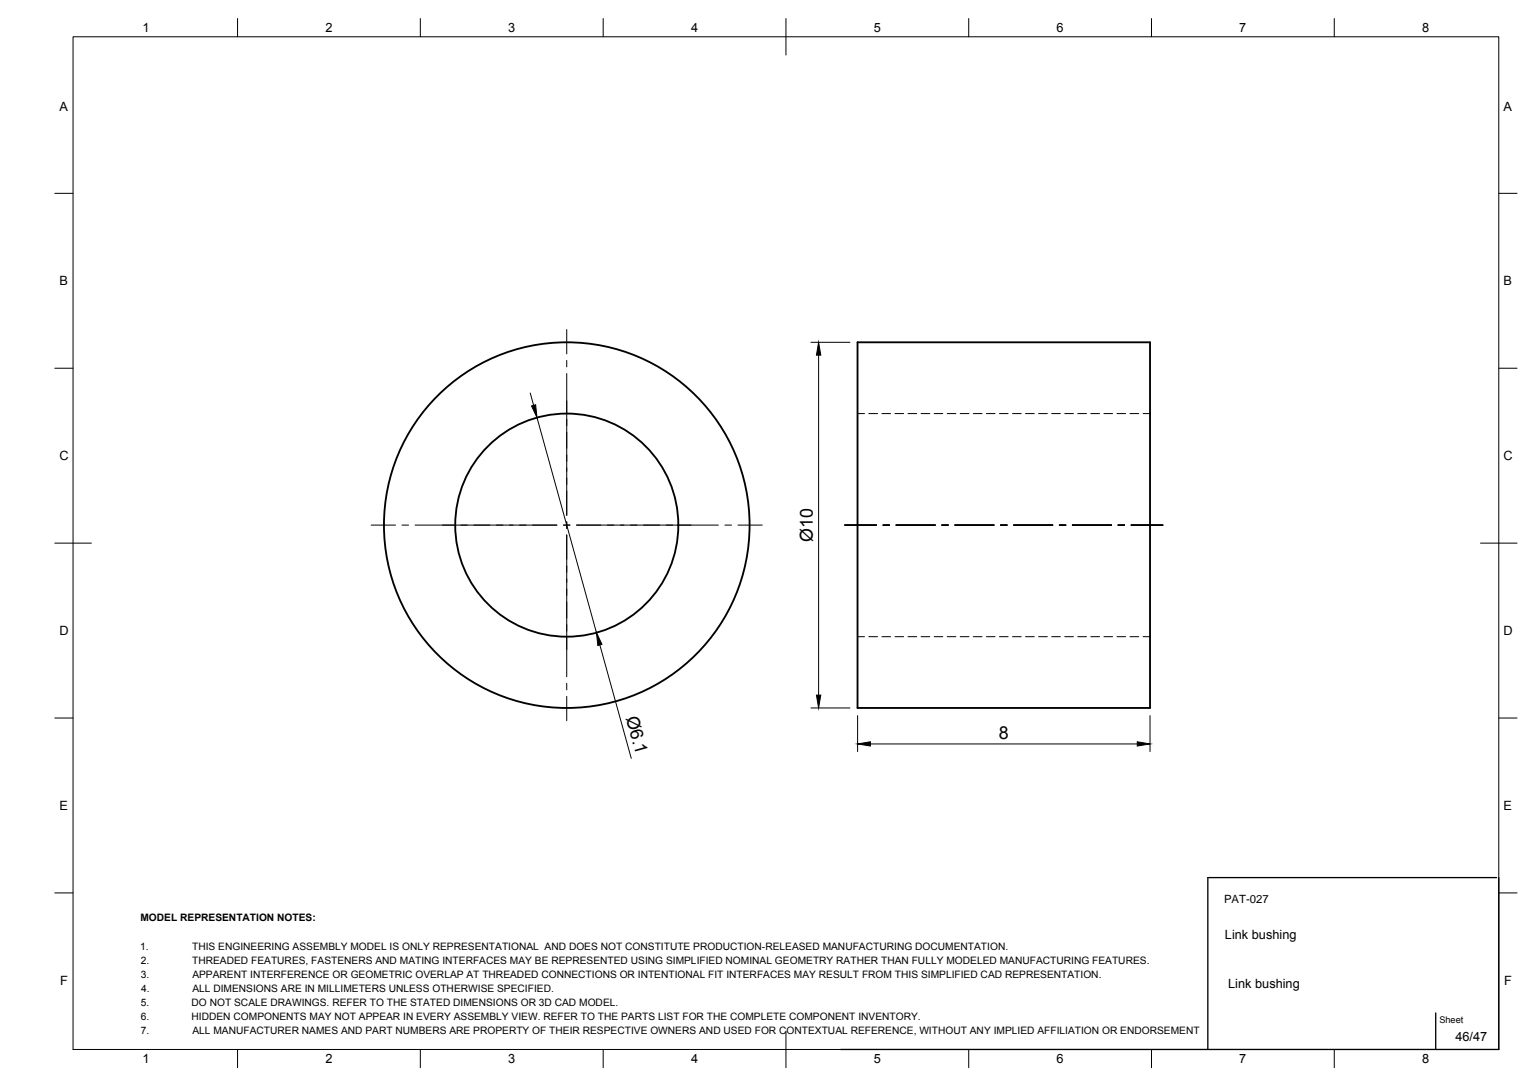
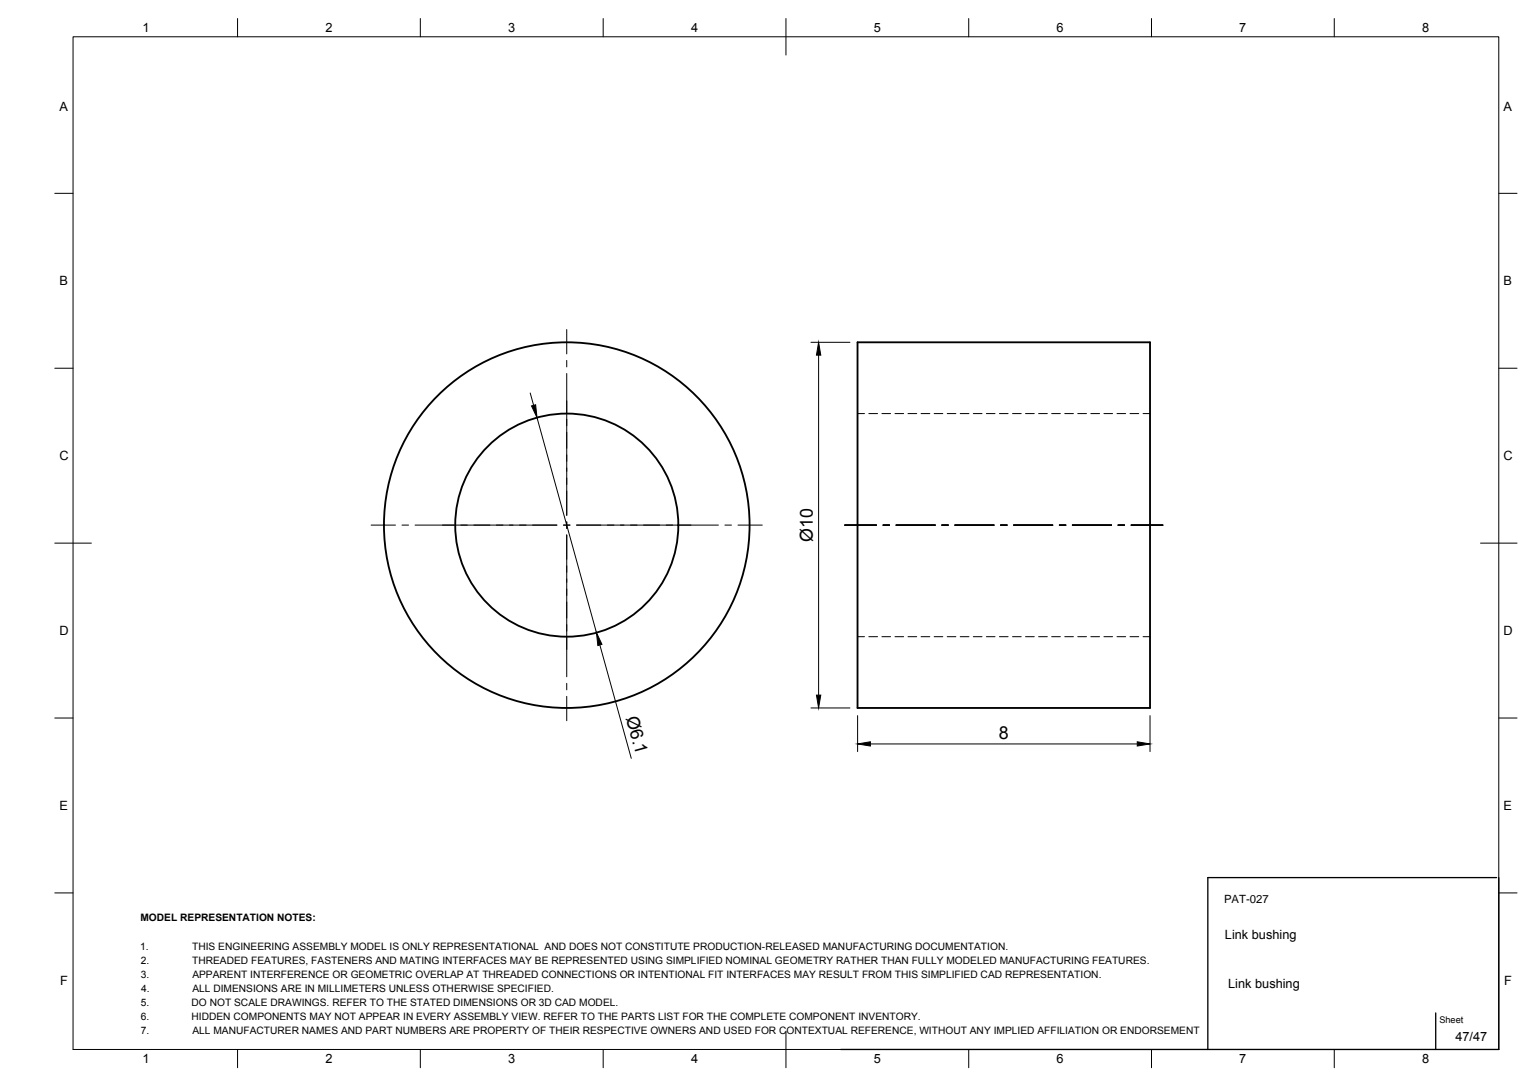
ISO-10303-21;
HEADER;
/* Generated by software containing ST-Developer
 * from STEP Tools, Inc. (www.steptools.com) 
 */

FILE_DESCRIPTION(
/* description */ ('Crank-driven oscillating fan base (mechanism only)'),

/* implementation_level */ '2;1');

FILE_NAME(
/* name */ 'Link bushing.step',
/* time_stamp */ '2026-10-28T03:25:00-07:00',
/* author */ (''),
/* organization */ (''),
/* preprocessor_version */ 'ST-DEVELOPER v20.2',
/* originating_system */ 'Autodesk Translation Framework v15.17.0.0',
/* authorisation */ '');

FILE_SCHEMA (('AUTOMOTIVE_DESIGN { 1 0 10303 214 3 1 1 }'));
ENDSEC;

DATA;
#10=MECHANICAL_DESIGN_GEOMETRIC_PRESENTATION_REPRESENTATION('',(#483),#11916);
#395=SHAPE_REPRESENTATION_RELATIONSHIP('SRR','None',#12123,#435);
#435=ADVANCED_BREP_SHAPE_REPRESENTATION('',(#528),#11914);
#483=STYLED_ITEM('',(#12361),#528);
#528=MANIFOLD_SOLID_BREP('Body1',#6116);
#688=FACE_BOUND('',#1789,.T.);
#689=FACE_BOUND('',#1791,.T.);
#882=PLANE('',#7393);
#883=PLANE('',#7394);
#1253=FACE_OUTER_BOUND('',#1786,.T.);
#1254=FACE_OUTER_BOUND('',#1787,.T.);
#1255=FACE_OUTER_BOUND('',#1788,.T.);
#1256=FACE_OUTER_BOUND('',#1790,.T.);
#1786=EDGE_LOOP('',(#5522,#5523,#5524,#5525));
#1787=EDGE_LOOP('',(#5526,#5527,#5528,#5529));
#1788=EDGE_LOOP('',(#5530));
#1789=EDGE_LOOP('',(#5531));
#1790=EDGE_LOOP('',(#5532));
#1791=EDGE_LOOP('',(#5533));
#2127=LINE('',#11791,#2460);
#2128=LINE('',#11797,#2461);
#2460=VECTOR('',#9400,0.305);
#2461=VECTOR('',#9407,0.5);
#2821=CIRCLE('',#7388,0.305);
#2822=CIRCLE('',#7389,0.305);
#2823=CIRCLE('',#7391,0.5);
#2824=CIRCLE('',#7392,0.5);
#3321=VERTEX_POINT('',#11788);
#3322=VERTEX_POINT('',#11790);
#3323=VERTEX_POINT('',#11794);
#3324=VERTEX_POINT('',#11796);
#4056=EDGE_CURVE('',#3321,#3321,#2821,.T.);
#4057=EDGE_CURVE('',#3321,#3322,#2127,.T.);
#4058=EDGE_CURVE('',#3322,#3322,#2822,.T.);
#4059=EDGE_CURVE('',#3323,#3323,#2823,.T.);
#4060=EDGE_CURVE('',#3323,#3324,#2128,.T.);
#4061=EDGE_CURVE('',#3324,#3324,#2824,.T.);
#5522=ORIENTED_EDGE('',*,*,#4056,.F.);
#5523=ORIENTED_EDGE('',*,*,#4057,.T.);
#5524=ORIENTED_EDGE('',*,*,#4058,.T.);
#5525=ORIENTED_EDGE('',*,*,#4057,.F.);
#5526=ORIENTED_EDGE('',*,*,#4059,.F.);
#5527=ORIENTED_EDGE('',*,*,#4060,.T.);
#5528=ORIENTED_EDGE('',*,*,#4061,.T.);
#5529=ORIENTED_EDGE('',*,*,#4060,.F.);
#5530=ORIENTED_EDGE('',*,*,#4059,.T.);
#5531=ORIENTED_EDGE('',*,*,#4056,.T.);
#5532=ORIENTED_EDGE('',*,*,#4061,.F.);
#5533=ORIENTED_EDGE('',*,*,#4058,.F.);
#5688=CYLINDRICAL_SURFACE('',#7387,0.305);
#5689=CYLINDRICAL_SURFACE('',#7390,0.5);
#6059=ADVANCED_FACE('',(#1253),#5688,.F.);
#6060=ADVANCED_FACE('',(#1254),#5689,.T.);
#6061=ADVANCED_FACE('',(#1255,#688),#882,.T.);
#6062=ADVANCED_FACE('',(#1256,#689),#883,.F.);
#6116=CLOSED_SHELL('',(#6059,#6060,#6061,#6062));
#7386=AXIS2_PLACEMENT_3D('',#11786,#9394,#9395);
#7387=AXIS2_PLACEMENT_3D('',#11787,#9396,#9397);
#7388=AXIS2_PLACEMENT_3D('',#11789,#9398,#9399);
#7389=AXIS2_PLACEMENT_3D('',#11792,#9401,#9402);
#7390=AXIS2_PLACEMENT_3D('',#11793,#9403,#9404);
#7391=AXIS2_PLACEMENT_3D('',#11795,#9405,#9406);
#7392=AXIS2_PLACEMENT_3D('',#11798,#9408,#9409);
#7393=AXIS2_PLACEMENT_3D('',#11799,#9410,#9411);
#7394=AXIS2_PLACEMENT_3D('',#11800,#9412,#9413);
#9394=DIRECTION('axis',(0.,0.,1.));
#9395=DIRECTION('refdir',(1.,0.,0.));
#9396=DIRECTION('center_axis',(0.,0.,1.));
#9397=DIRECTION('ref_axis',(1.,0.,0.));
#9398=DIRECTION('center_axis',(0.,0.,-1.));
#9399=DIRECTION('ref_axis',(1.,0.,0.));
#9400=DIRECTION('',(0.,0.,-1.));
#9401=DIRECTION('center_axis',(0.,0.,-1.));
#9402=DIRECTION('ref_axis',(1.,0.,0.));
#9403=DIRECTION('center_axis',(0.,0.,1.));
#9404=DIRECTION('ref_axis',(1.,0.,0.));
#9405=DIRECTION('center_axis',(0.,0.,1.));
#9406=DIRECTION('ref_axis',(1.,0.,0.));
#9407=DIRECTION('',(0.,0.,-1.));
#9408=DIRECTION('center_axis',(0.,0.,1.));
#9409=DIRECTION('ref_axis',(1.,0.,0.));
#9410=DIRECTION('center_axis',(0.,0.,1.));
#9411=DIRECTION('ref_axis',(1.,0.,0.));
#9412=DIRECTION('center_axis',(0.,0.,1.));
#9413=DIRECTION('ref_axis',(1.,0.,0.));
#11786=CARTESIAN_POINT('',(0.,0.,0.));
#11787=CARTESIAN_POINT('Origin',(-0.429855350392604,2.61349944954989,8.6));
#11788=CARTESIAN_POINT('',(-0.734855350392604,2.61349944954989,9.4));
#11789=CARTESIAN_POINT('Origin',(-0.429855350392604,2.61349944954989,9.4));
#11790=CARTESIAN_POINT('',(-0.734855350392604,2.61349944954989,8.6));
#11791=CARTESIAN_POINT('',(-0.734855350392604,2.61349944954989,8.6));
#11792=CARTESIAN_POINT('Origin',(-0.429855350392604,2.61349944954989,8.6));
#11793=CARTESIAN_POINT('Origin',(-0.429855350392604,2.61349944954989,8.6));
#11794=CARTESIAN_POINT('',(-0.929855350392604,2.61349944954989,9.4));
#11795=CARTESIAN_POINT('Origin',(-0.429855350392604,2.61349944954989,9.4));
#11796=CARTESIAN_POINT('',(-0.929855350392604,2.61349944954989,8.6));
#11797=CARTESIAN_POINT('',(-0.929855350392604,2.61349944954989,8.6));
#11798=CARTESIAN_POINT('Origin',(-0.429855350392604,2.61349944954989,8.6));
#11799=CARTESIAN_POINT('Origin',(-0.429855350392604,2.61349944954989,9.4));
#11800=CARTESIAN_POINT('Origin',(-0.429855350392604,2.61349944954989,8.6));
#11867=UNCERTAINTY_MEASURE_WITH_UNIT(LENGTH_MEASURE(0.001),#11917,
'DISTANCE_ACCURACY_VALUE',
'Maximum model space distance between geometric entities at asserted c
onnectivities');
#11869=UNCERTAINTY_MEASURE_WITH_UNIT(LENGTH_MEASURE(0.001),#11917,
'DISTANCE_ACCURACY_VALUE',
'Maximum model space distance between geometric entities at asserted c
onnectivities');
#11914=(
GEOMETRIC_REPRESENTATION_CONTEXT(3)
GLOBAL_UNCERTAINTY_ASSIGNED_CONTEXT((#11867))
GLOBAL_UNIT_ASSIGNED_CONTEXT((#11917,#11919,#11920))
REPRESENTATION_CONTEXT('','3D')
);
#11916=(
GEOMETRIC_REPRESENTATION_CONTEXT(3)
GLOBAL_UNCERTAINTY_ASSIGNED_CONTEXT((#11869))
GLOBAL_UNIT_ASSIGNED_CONTEXT((#11917,#11919,#11920))
REPRESENTATION_CONTEXT('','3D')
);
#11917=(
LENGTH_UNIT()
NAMED_UNIT(*)
SI_UNIT(.CENTI.,.METRE.)
);
#11919=(
NAMED_UNIT(*)
PLANE_ANGLE_UNIT()
SI_UNIT($,.RADIAN.)
);
#11920=(
NAMED_UNIT(*)
SI_UNIT($,.STERADIAN.)
SOLID_ANGLE_UNIT()
);
#11965=SHAPE_DEFINITION_REPRESENTATION(#12070,#12123);
#12070=PRODUCT_DEFINITION_SHAPE('',$,#12170);
#12123=SHAPE_REPRESENTATION('',(#7386),#11914);
#12125=PRODUCT_DEFINITION_CONTEXT('part definition',#12265,'design');
#12170=PRODUCT_DEFINITION('Link bushing','Link bushing',#12216,#12125);
#12216=PRODUCT_DEFINITION_FORMATION('',$,#12311);
#12265=APPLICATION_CONTEXT(
'Core Data for Automotive Mechanical Design Process');
#12266=PRODUCT_CONTEXT('part definition',#12265,'mechanical');
#12311=PRODUCT('Link bushing','Link bushing','Link bushing',(#12266));
#12355=COLOUR_RGB('Light Blue',0.38,0.62,0.78);
#12356=FILL_AREA_STYLE_COLOUR('',#12355);
#12357=FILL_AREA_STYLE('',(#12356));
#12358=SURFACE_STYLE_FILL_AREA(#12357);
#12359=SURFACE_SIDE_STYLE('',(#12358));
#12360=SURFACE_STYLE_USAGE(.BOTH.,#12359);
#12361=PRESENTATION_STYLE_ASSIGNMENT((#12360));
ENDSEC;
END-ISO-10303-21;
